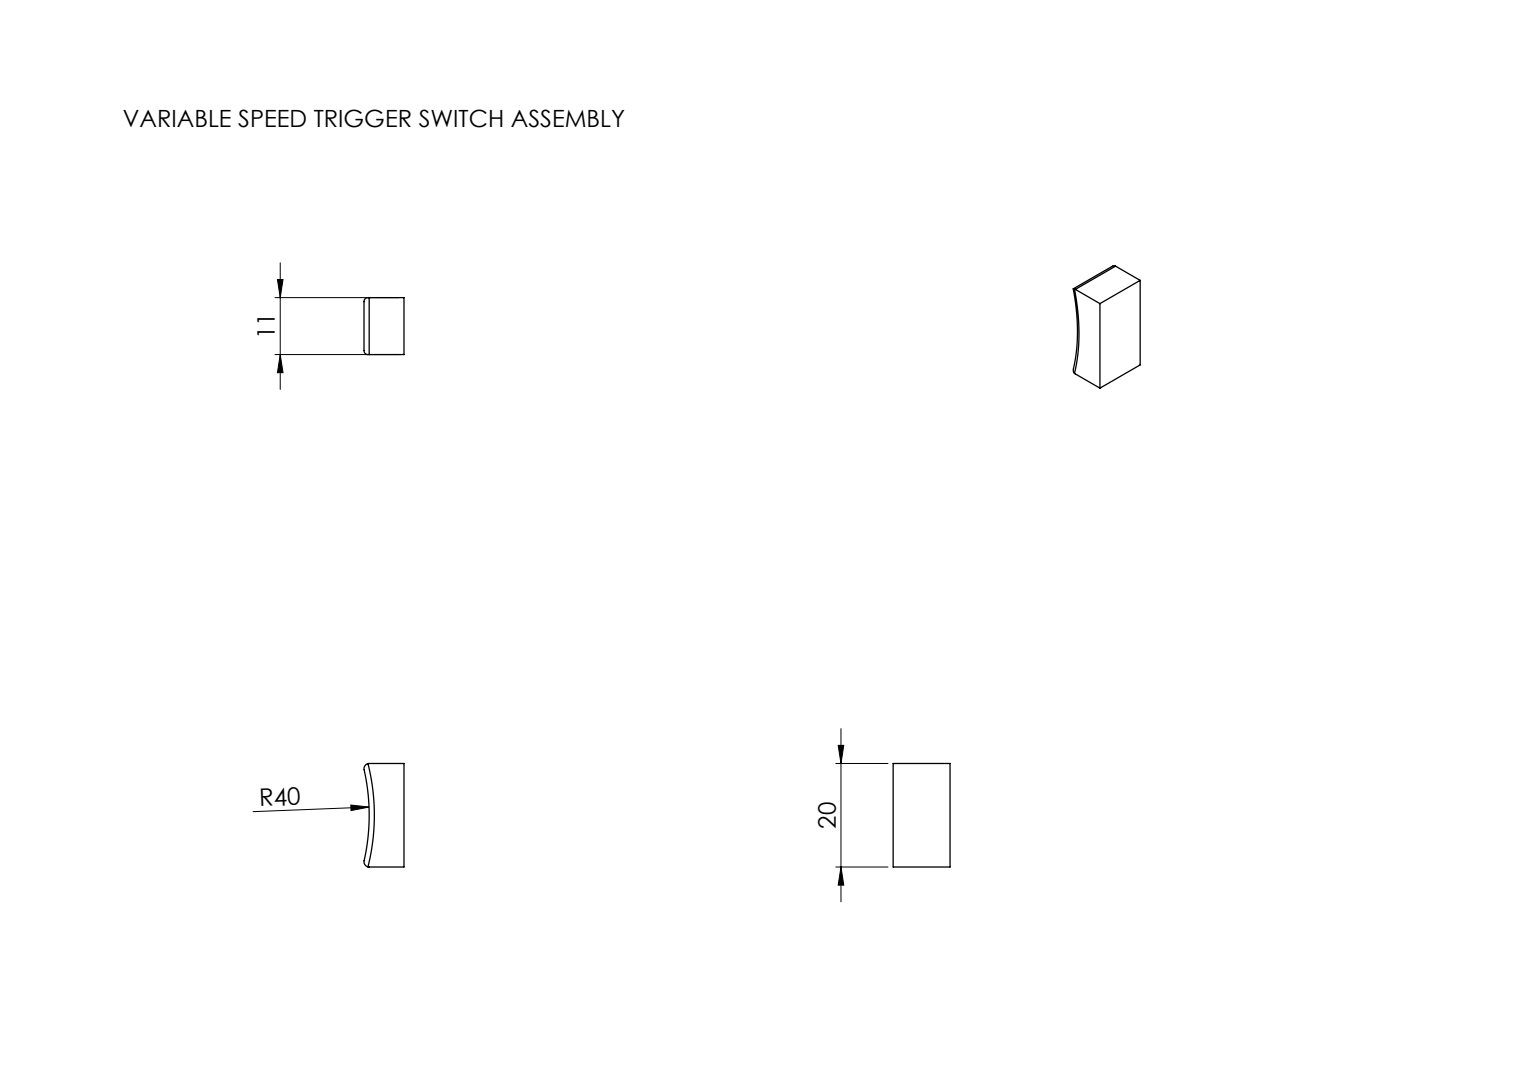
ISO-10303-21;
HEADER;
FILE_DESCRIPTION (('STEP AP214'),
    '1' );
FILE_NAME ('Variable Speed Trigger Switch assembly.step',
    '2026-10-05T20:22:16',
    ( '' ),
    ( '' ),
    'SwSTEP 2.0',
    'SolidWorks 2026',
    '' );
FILE_SCHEMA (( 'AUTOMOTIVE_DESIGN' ));
ENDSEC;

DATA;
#2=EDGE_CURVE ( 'NONE', #9188, #6176, #1844, .T. ) ;
#111=LINE ( 'NONE', #8166, #1932 ) ;
#145=DIRECTION ( 'NONE',  ( 0.000000000000000000, -0.000000000000000000, -1.000000000000000000 ) ) ;
#155=EDGE_CURVE ( 'NONE', #4227, #5635, #15763, .T. ) ;
#178=ORIENTED_EDGE ( 'NONE', *, *, #2632, .F. ) ;
#200=AXIS2_PLACEMENT_3D ( 'NONE', #10939, #4055, #145 ) ;
#265=DIRECTION ( 'NONE',  ( -0.000000000000000000, -0.000000000000000000, -1.000000000000000000 ) ) ;
#273=VECTOR ( 'NONE', #8822, 1000.000000000000000 ) ;
#311=CARTESIAN_POINT ( 'NONE',  ( -32.66708739526796279, 119.0000000000141824, -4.722170599054655860 ) ) ;
#314=CARTESIAN_POINT ( 'NONE',  ( -31.89848094669885725, 100.0271397714182342, 5.500000000000000000 ) ) ;
#331=CARTESIAN_POINT ( 'NONE',  ( -31.66708739526795924, 120.0000000000000284, -5.500000000000000000 ) ) ;
#383=DIRECTION ( 'NONE',  ( 3.469446951953614189E-16, -1.000000000000000000, 0.000000000000000000 ) ) ;
#427=VECTOR ( 'NONE', #13768, 1000.000000000000000 ) ;
#450=CARTESIAN_POINT ( 'NONE',  ( -32.02886766642249228, 119.9418479153533781, 5.500000000000000888 ) ) ;
#462=ORIENTED_EDGE ( 'NONE', *, *, #5545, .F. ) ;
#521=FILL_AREA_STYLE_COLOUR ( '', #2206 ) ;
#528=ORIENTED_EDGE ( 'NONE', *, *, #5545, .T. ) ;
#601=B_SPLINE_CURVE_WITH_KNOTS ( 'NONE', 3,
 ( #15955, #13311, #9052, #1176 ),
 .UNSPECIFIED., .F., .F.,
 ( 4, 4 ),
 ( -6.324563032106999871E-06, 0.0003067249959486805411 ),
 .UNSPECIFIED. ) ;
#623=EDGE_CURVE ( 'NONE', #8295, #4586, #6392, .T. ) ;
#656=CYLINDRICAL_SURFACE ( 'NONE', #15299, 1.000000000000000888 ) ;
#696=( LENGTH_UNIT ( ) NAMED_UNIT ( * ) SI_UNIT ( .MILLI., .METRE. ) );
#733=CARTESIAN_POINT ( 'NONE',  ( -32.64269715136552463, 118.7804878048780779, 4.500000000000000000 ) ) ;
#764=ORIENTED_EDGE ( 'NONE', *, *, #8937, .T. ) ;
#782=ADVANCED_FACE ( 'NONE', ( #2094 ), #7493, .T. ) ;
#907=CARTESIAN_POINT ( 'NONE',  ( -32.66708739526796279, 119.0000000000000284, 4.722170599040653727 ) ) ;
#1034=( NAMED_UNIT ( * ) SI_UNIT ( $, .STERADIAN. ) SOLID_ANGLE_UNIT ( ) );
#1168=DIRECTION ( 'NONE',  ( -1.000000000000000000, 0.000000000000000000, 0.000000000000000000 ) ) ;
#1176=CARTESIAN_POINT ( 'NONE',  ( -32.66708739526796279, 101.0000000000000142, 4.722170599040663497 ) ) ;
#1214=ADVANCED_FACE ( 'NONE', ( #11195 ), #11869, .T. ) ;
#1336=CARTESIAN_POINT ( 'NONE',  ( -71.66708739526794147, 110.0000000000000142, -4.499999999999999112 ) ) ;
#1469=VECTOR ( 'NONE', #5604, 1000.000000000000000 ) ;
#1494=PRODUCT ( 'Variable Speed Trigger Switch assembly', 'Variable Speed Trigger Switch assembly', '', ( #6686 ) ) ;
#1500=CARTESIAN_POINT ( 'NONE',  ( -32.59761674097325823, 119.3792650757663978, -5.080178642870992967 ) ) ;
#1501=CARTESIAN_POINT ( 'NONE',  ( -71.66708739526794147, 110.0000000000000142, -5.500000000000000000 ) ) ;
#1570=DIRECTION ( 'NONE',  ( 0.000000000000000000, 0.000000000000000000, 1.000000000000000000 ) ) ;
#1620=STYLED_ITEM ( 'NONE', ( #7941 ), #16900 ) ;
#1644=CARTESIAN_POINT ( 'NONE',  ( -32.02886766642248517, 100.0581520846466930, 5.500000000000000000 ) ) ;
#1692=ORIENTED_EDGE ( 'NONE', *, *, #9652, .F. ) ;
#1792=EDGE_LOOP ( 'NONE', ( #8992, #15963, #14025, #11089 ) ) ;
#1840=ORIENTED_EDGE ( 'NONE', *, *, #2784, .F. ) ;
#1842=EDGE_LOOP ( 'NONE', ( #6707, #13226, #11700, #4645 ) ) ;
#1844=B_SPLINE_CURVE_WITH_KNOTS ( 'NONE', 3,
 ( #8174, #11087, #2865, #16587 ),
 .UNSPECIFIED., .F., .F.,
 ( 4, 4 ),
 ( 0.001580575003428885293, 0.001893147295999754844 ),
 .UNSPECIFIED. ) ;
#1849=CARTESIAN_POINT ( 'NONE',  ( -31.66708739526795924, 119.0000000000000284, 5.500000000000000000 ) ) ;
#1853=AXIS2_PLACEMENT_3D ( 'NONE', #13518, #6796, #12191 ) ;
#1932=VECTOR ( 'NONE', #6853, 1000.000000000000000 ) ;
#1941=DIRECTION ( 'NONE',  ( -0.000000000000000000, -0.000000000000000000, -1.000000000000000000 ) ) ;
#1964=CARTESIAN_POINT ( 'NONE',  ( -32.14917720409752633, 119.8847850876495471, 5.472305571546614900 ) ) ;
#1979=EDGE_CURVE ( 'NONE', #5635, #9188, #7587, .T. ) ;
#2047=CARTESIAN_POINT ( 'NONE',  ( -31.66708739526795924, 101.0000000000000142, 5.500000000000000000 ) ) ;
#2094=FACE_OUTER_BOUND ( 'NONE', #9674, .T. ) ;
#2099=( NAMED_UNIT ( * ) SI_UNIT ( $, .STERADIAN. ) SOLID_ANGLE_UNIT ( ) );
#2113=VECTOR ( 'NONE', #4048, 1000.000000000000000 ) ;
#2140=CIRCLE ( 'NONE', #1853, 39.99999999999997868 ) ;
#2144=VERTEX_POINT ( 'NONE', #4204 ) ;
#2186=DIRECTION ( 'NONE',  ( -0.000000000000000000, -0.000000000000000000, -1.000000000000000000 ) ) ;
#2206=COLOUR_RGB ( '', 0.40784314, 0.44705882, 0.49803922) ;
#2370=PLANE ( 'NONE',  #14682 ) ;
#2381=CARTESIAN_POINT ( 'NONE',  ( -31.89848094669885725, 100.0271397714182342, -5.500000000000000000 ) ) ;
#2404=ORIENTED_EDGE ( 'NONE', *, *, #2, .F. ) ;
#2580=APPLICATION_CONTEXT ( 'automotive_design' ) ;
#2629=ORIENTED_EDGE ( 'NONE', *, *, #12849, .F. ) ;
#2632=EDGE_CURVE ( 'NONE', #7206, #9188, #16191, .T. ) ;
#2668=CARTESIAN_POINT ( 'NONE',  ( -71.66708739526794147, 110.0000000000000142, 4.500000000000000000 ) ) ;
#2744=CARTESIAN_POINT ( 'NONE',  ( -32.34996859904739352, 119.7408970890944744, -5.378151393595213214 ) ) ;
#2759=DIRECTION ( 'NONE',  ( 0.000000000000000000, 0.000000000000000000, 1.000000000000000000 ) ) ;
#2784=EDGE_CURVE ( 'NONE', #15700, #10662, #3443, .T. ) ;
#2785=ORIENTED_EDGE ( 'NONE', *, *, #1979, .T. ) ;
#2828=CARTESIAN_POINT ( 'NONE',  ( -32.66708739526796279, 119.0000000000141824, -4.722170599054655860 ) ) ;
#2833=DIRECTION ( 'NONE',  ( -1.000000000000000000, 0.000000000000000000, 0.000000000000000000 ) ) ;
#2865=CARTESIAN_POINT ( 'NONE',  ( -32.65876937324898677, 118.8519199021378938, -4.574127464417287570 ) ) ;
#2958=DIRECTION ( 'NONE',  ( -0.000000000000000000, -0.000000000000000000, -1.000000000000000000 ) ) ;
#3083=DIRECTION ( 'NONE',  ( -1.000000000000000000, 0.000000000000000000, 0.000000000000000000 ) ) ;
#3159=ORIENTED_EDGE ( 'NONE', *, *, #12950, .T. ) ;
#3179=( NAMED_UNIT ( * ) SI_UNIT ( $, .STERADIAN. ) SOLID_ANGLE_UNIT ( ) );
#3275=VERTEX_POINT ( 'NONE', #3762 ) ;
#3285=EDGE_CURVE ( 'NONE', #4393, #17452, #16707, .T. ) ;
#3290=LINE ( 'NONE', #14101, #1469 ) ;
#3291=CARTESIAN_POINT ( 'NONE',  ( -32.34996859905196231, 119.7408970890905096, 5.378151393592371043 ) ) ;
#3303=ORIENTED_EDGE ( 'NONE', *, *, #6295, .T. ) ;
#3441=SURFACE_SIDE_STYLE ('',( #15381 ) ) ;
#3443=LINE ( 'NONE', #14238, #11031 ) ;
#3473=CARTESIAN_POINT ( 'NONE',  ( -32.66708739526796279, 118.9256726598784866, 4.648823768412006174 ) ) ;
#3475=VERTEX_POINT ( 'NONE', #11444 ) ;
#3476=ADVANCED_FACE ( 'NONE', ( #11180 ), #16854, .F. ) ;
#3480=ORIENTED_EDGE ( 'NONE', *, *, #10562, .F. ) ;
#3518=CARTESIAN_POINT ( 'NONE',  ( -32.66708739526796279, 119.0000000000000284, 5.500000000000000000 ) ) ;
#3583=AXIS2_PLACEMENT_3D ( 'NONE', #5482, #6893, #8222 ) ;
#3762=CARTESIAN_POINT ( 'NONE',  ( -24.93725393319378725, 100.0000000000000142, 5.500000000000000000 ) ) ;
#3768=CARTESIAN_POINT ( 'NONE',  ( -32.66708739526796279, 101.0000000000000142, -4.722170599040662609 ) ) ;
#3776=FILL_AREA_STYLE_COLOUR ( '', #15186 ) ;
#3789=UNCERTAINTY_MEASURE_WITH_UNIT (LENGTH_MEASURE( 1.000000000000000082E-05 ), #696, 'distance_accuracy_value', 'NONE');
#3800=EDGE_CURVE ( 'NONE', #17452, #7206, #7303, .T. ) ;
#3887=( GEOMETRIC_REPRESENTATION_CONTEXT ( 3 ) GLOBAL_UNCERTAINTY_ASSIGNED_CONTEXT ( ( #17305 ) ) GLOBAL_UNIT_ASSIGNED_CONTEXT ( ( #11826, #10317, #1034 ) ) REPRESENTATION_CONTEXT ( 'NONE', 'WORKASPACE' ) );
#3915=ORIENTED_EDGE ( 'NONE', *, *, #623, .T. ) ;
#3973=CARTESIAN_POINT ( 'NONE',  ( -32.43085388486576193, 100.3453498474263910, -5.312352690998809912 ) ) ;
#4048=DIRECTION ( 'NONE',  ( -1.000000000000000000, -0.000000000000000000, -0.000000000000000000 ) ) ;
#4055=DIRECTION ( 'NONE',  ( 0.000000000000000000, -1.000000000000000000, 0.000000000000000000 ) ) ;
#4103=CARTESIAN_POINT ( 'NONE',  ( -31.89848094669886436, 119.9728602285818084, -5.500000000000000000 ) ) ;
#4117=CARTESIAN_POINT ( 'NONE',  ( -32.66708739526796279, 119.0000000000000284, 4.722170599040653727 ) ) ;
#4204=CARTESIAN_POINT ( 'NONE',  ( -24.93725393319379435, 120.0000000000000284, -5.500000000000000000 ) ) ;
#4227=VERTEX_POINT ( 'NONE', #7143 ) ;
#4249=CARTESIAN_POINT ( 'NONE',  ( -32.55406425504222057, 119.4745293701363664, -5.163900856529947347 ) ) ;
#4276=CARTESIAN_POINT ( 'NONE',  ( -32.64269715136552463, 118.7804878048780779, -4.499999999999999112 ) ) ;
#4297=CARTESIAN_POINT ( 'NONE',  ( -71.66708739526794147, 110.0000000000000142, 5.500000000000000000 ) ) ;
#4322=LINE ( 'NONE', #13700, #7340 ) ;
#4324=CARTESIAN_POINT ( 'NONE',  ( -32.64269715136552463, 101.2195121951219647, -4.499999999999999112 ) ) ;
#4332=DIRECTION ( 'NONE',  ( 0.000000000000000000, 0.000000000000000000, 1.000000000000000000 ) ) ;
#4379=DIRECTION ( 'NONE',  ( -0.000000000000000000, -0.000000000000000000, -1.000000000000000000 ) ) ;
#4393=VERTEX_POINT ( 'NONE', #11387 ) ;
#4452=CARTESIAN_POINT ( 'NONE',  ( -32.66708739526796279, 119.0000000000000284, 4.722170599040653727 ) ) ;
#4475=CARTESIAN_POINT ( 'NONE',  ( -31.66708739526795924, 101.0000000000000142, 5.500000000000000000 ) ) ;
#4477=PRODUCT_DEFINITION_SHAPE ( 'NONE', 'NONE',  #5120 ) ;
#4508=CARTESIAN_POINT ( 'NONE',  ( -71.66708739526794147, 110.0000000000000142, -5.500000000000000000 ) ) ;
#4586=VERTEX_POINT ( 'NONE', #9419 ) ;
#4627=CARTESIAN_POINT ( 'NONE',  ( -32.43085388486576193, 119.6546501525736375, 5.312352690998810800 ) ) ;
#4645=ORIENTED_EDGE ( 'NONE', *, *, #8937, .F. ) ;
#4727=VECTOR ( 'NONE', #265, 1000.000000000000000 ) ;
#4734=ORIENTED_EDGE ( 'NONE', *, *, #12950, .F. ) ;
#4735=CARTESIAN_POINT ( 'NONE',  ( -32.43085388486576903, 100.3453498474263768, 5.312352690998809024 ) ) ;
#4772=SHAPE_REPRESENTATION_RELATIONSHIP ( 'NONE' , 'NONE' ,  #13460, #10572 ) ;
#4829=AXIS2_PLACEMENT_3D ( 'NONE', #11999, #14921, #8191 ) ;
#4833=AXIS2_PLACEMENT_3D ( 'NONE', #14393, #17123, #5002 ) ;
#4933=DIRECTION ( 'NONE',  ( -0.000000000000000000, -0.000000000000000000, -1.000000000000000000 ) ) ;
#4972=CARTESIAN_POINT ( 'NONE',  ( -71.66708739526794147, 110.0000000000000142, 4.500000000000000000 ) ) ;
#5002=DIRECTION ( 'NONE',  ( -1.000000000000000000, 0.000000000000000000, 0.000000000000000000 ) ) ;
#5009=LINE ( 'NONE', #17132, #2113 ) ;
#5018=CARTESIAN_POINT ( 'NONE',  ( -31.89848094669885725, 100.0271397714182342, -5.500000000000000000 ) ) ;
#5120=PRODUCT_DEFINITION ( 'UNKNOWN', '', #12096, #9369 ) ;
#5288=SURFACE_STYLE_FILL_AREA ( #6263 ) ;
#5482=CARTESIAN_POINT ( 'NONE',  ( 0.000000000000000000, 0.000000000000000000, 0.000000000000000000 ) ) ;
#5515=EDGE_LOOP ( 'NONE', ( #5570, #16193, #16050, #7766, #14975, #16631 ) ) ;
#5545=EDGE_CURVE ( 'NONE', #17341, #4393, #12084, .T. ) ;
#5570=ORIENTED_EDGE ( 'NONE', *, *, #6017, .T. ) ;
#5604=DIRECTION ( 'NONE',  ( 1.000000000000000000, -0.000000000000000000, -0.000000000000000000 ) ) ;
#5635=VERTEX_POINT ( 'NONE', #4117 ) ;
#5638=ADVANCED_FACE ( 'NONE', ( #6784 ), #8350, .F. ) ;
#5713=DIRECTION ( 'NONE',  ( -1.000000000000000000, 0.000000000000000000, 0.000000000000000000 ) ) ;
#5725=ORIENTED_EDGE ( 'NONE', *, *, #8449, .T. ) ;
#5741=ORIENTED_EDGE ( 'NONE', *, *, #3800, .F. ) ;
#5780=VECTOR ( 'NONE', #8506, 1000.000000000000000 ) ;
#5782=CARTESIAN_POINT ( 'NONE',  ( -31.66708739526795924, 100.0000000000000142, 5.500000000000000000 ) ) ;
#5836=DIRECTION ( 'NONE',  ( -1.000000000000000000, 0.000000000000000000, 0.000000000000000000 ) ) ;
#5845=DIRECTION ( 'NONE',  ( -0.000000000000000000, -0.000000000000000000, -1.000000000000000000 ) ) ;
#5855=CARTESIAN_POINT ( 'NONE',  ( -32.66708739526796279, 101.0000000000000142, -4.722170599040662609 ) ) ;
#5859=TOROIDAL_SURFACE ( 'NONE', #8394, 40.99999999999998579, 1.000000000000000000 ) ;
#5902=ORIENTED_EDGE ( 'NONE', *, *, #3800, .T. ) ;
#5952=CARTESIAN_POINT ( 'NONE',  ( -32.64269715136552463, 101.2195121951219647, -4.499999999999999112 ) ) ;
#5980=CARTESIAN_POINT ( 'NONE',  ( -32.59761674097720174, 100.6207349242430809, 5.080178642862614780 ) ) ;
#6009=( LENGTH_UNIT ( ) NAMED_UNIT ( * ) SI_UNIT ( .MILLI., .METRE. ) );
#6017=EDGE_CURVE ( 'NONE', #11430, #3475, #601, .T. ) ;
#6111=ORIENTED_EDGE ( 'NONE', *, *, #8449, .F. ) ;
#6176=VERTEX_POINT ( 'NONE', #4276 ) ;
#6263=FILL_AREA_STYLE ('',( #3776 ) ) ;
#6265=EDGE_LOOP ( 'NONE', ( #8080, #14588, #3915, #3303, #5725, #8757 ) ) ;
#6295=EDGE_CURVE ( 'NONE', #4586, #17341, #14879, .T. ) ;
#6315=EDGE_LOOP ( 'NONE', ( #5902, #3159, #9035, #3480, #1692, #16838 ) ) ;
#6392=CIRCLE ( 'NONE', #7530, 40.99999999999997868 ) ;
#6499=ORIENTED_EDGE ( 'NONE', *, *, #6295, .F. ) ;
#6531=CARTESIAN_POINT ( 'NONE',  ( -32.14917720409751922, 100.1152149123505239, -5.472305571546616676 ) ) ;
#6638=VERTEX_POINT ( 'NONE', #8574 ) ;
#6640=CARTESIAN_POINT ( 'NONE',  ( -32.14917720409452073, 119.8847850876509966, -5.472305571547330771 ) ) ;
#6686=PRODUCT_CONTEXT ( 'NONE', #7328, 'mechanical' ) ;
#6707=ORIENTED_EDGE ( 'NONE', *, *, #14410, .F. ) ;
#6752=EDGE_CURVE ( 'NONE', #10662, #8295, #8594, .T. ) ;
#6784=FACE_OUTER_BOUND ( 'NONE', #14962, .T. ) ;
#6791=ORIENTED_EDGE ( 'NONE', *, *, #2, .T. ) ;
#6796=DIRECTION ( 'NONE',  ( -0.000000000000000000, -0.000000000000000000, -1.000000000000000000 ) ) ;
#6827=DIRECTION ( 'NONE',  ( -0.000000000000000000, -0.000000000000000000, -1.000000000000000000 ) ) ;
#6853=DIRECTION ( 'NONE',  ( -1.000000000000000000, -0.000000000000000000, -0.000000000000000000 ) ) ;
#6893=DIRECTION ( 'NONE',  ( 0.000000000000000000, 0.000000000000000000, 1.000000000000000000 ) ) ;
#6990=FACE_OUTER_BOUND ( 'NONE', #17295, .T. ) ;
#7054=CIRCLE ( 'NONE', #16949, 39.99999999999997868 ) ;
#7143=CARTESIAN_POINT ( 'NONE',  ( -32.64269715136552463, 118.7804878048780779, 4.500000000000000000 ) ) ;
#7169=ORIENTED_EDGE ( 'NONE', *, *, #11708, .F. ) ;
#7206=VERTEX_POINT ( 'NONE', #4103 ) ;
#7245=AXIS2_PLACEMENT_3D ( 'NONE', #2047, #7440, #12841 ) ;
#7250=DIRECTION ( 'NONE',  ( -1.000000000000000000, 0.000000000000000000, 0.000000000000000000 ) ) ;
#7298=CARTESIAN_POINT ( 'NONE',  ( -32.66708739526796279, 101.0000000000000142, 4.722170599040663497 ) ) ;
#7303=CIRCLE ( 'NONE', #14648, 40.99999999999997868 ) ;
#7328=APPLICATION_CONTEXT ( 'automotive_design' ) ;
#7340=VECTOR ( 'NONE', #1570, 1000.000000000000000 ) ;
#7402=ORIENTED_EDGE ( 'NONE', *, *, #16890, .T. ) ;
#7405=EDGE_CURVE ( 'NONE', #5635, #8295, #9583, .T. ) ;
#7440=DIRECTION ( 'NONE',  ( 0.000000000000000000, 0.000000000000000000, 1.000000000000000000 ) ) ;
#7493=CYLINDRICAL_SURFACE ( 'NONE', #13015, 1.000000000000000888 ) ;
#7530=AXIS2_PLACEMENT_3D ( 'NONE', #8767, #5845, #12925 ) ;
#7540=CARTESIAN_POINT ( 'NONE',  ( -32.65879391391307252, 118.8520289717560843, 4.574240649589675911 ) ) ;
#7587=LINE ( 'NONE', #3518, #16113 ) ;
#7671=CARTESIAN_POINT ( 'NONE',  ( -32.02886766642249228, 100.0581520846466645, -5.500000000000001776 ) ) ;
#7766=ORIENTED_EDGE ( 'NONE', *, *, #7405, .F. ) ;
#7930=VECTOR ( 'NONE', #15717, 1000.000000000000000 ) ;
#7941=PRESENTATION_STYLE_ASSIGNMENT (( #11654 ) ) ;
#7977=DIRECTION ( 'NONE',  ( -0.000000000000000000, -0.000000000000000000, -1.000000000000000000 ) ) ;
#8080=ORIENTED_EDGE ( 'NONE', *, *, #14108, .T. ) ;
#8120=CARTESIAN_POINT ( 'NONE',  ( -24.93725393319378725, 100.0000000000000142, 5.500000000000000000 ) ) ;
#8149=CARTESIAN_POINT ( 'NONE',  ( -32.66708739526796279, 101.0000000000000142, 5.500000000000000000 ) ) ;
#8166=CARTESIAN_POINT ( 'NONE',  ( -32.93725393319379435, 120.0000000000000284, 5.500000000000000000 ) ) ;
#8174=CARTESIAN_POINT ( 'NONE',  ( -32.66708739526796279, 119.0000000000141824, -4.722170599054655860 ) ) ;
#8191=DIRECTION ( 'NONE',  ( -1.000000000000000000, 0.000000000000000000, 0.000000000000000000 ) ) ;
#8222=DIRECTION ( 'NONE',  ( 1.000000000000000000, 0.000000000000000000, 0.000000000000000000 ) ) ;
#8223=CARTESIAN_POINT ( 'NONE',  ( -32.66708739526662697, 119.0939651702628623, -4.814896201988002389 ) ) ;
#8295=VERTEX_POINT ( 'NONE', #9709 ) ;
#8350=CYLINDRICAL_SURFACE ( 'NONE', #13454, 39.99999999999997868 ) ;
#8358=CARTESIAN_POINT ( 'NONE',  ( -32.34996859905195521, 100.2591029109095189, 5.378151393592374596 ) ) ;
#8365=EDGE_LOOP ( 'NONE', ( #11702, #13362, #11371, #15316, #462, #6499 ) ) ;
#8394=AXIS2_PLACEMENT_3D ( 'NONE', #1336, #1941, #5836 ) ;
#8419=FACE_OUTER_BOUND ( 'NONE', #14217, .T. ) ;
#8449=EDGE_CURVE ( 'NONE', #17341, #3275, #11565, .T. ) ;
#8450=FACE_OUTER_BOUND ( 'NONE', #1842, .T. ) ;
#8500=AXIS2_PLACEMENT_3D ( 'NONE', #16574, #4933, #12671 ) ;
#8506=DIRECTION ( 'NONE',  ( -3.469446951953613696E-16, 1.000000000000000000, -0.000000000000000000 ) ) ;
#8574=CARTESIAN_POINT ( 'NONE',  ( -24.93725393319378725, 100.0000000000000142, -5.500000000000000000 ) ) ;
#8594=CIRCLE ( 'NONE', #8865, 1.000000000000000888 ) ;
#8604=ADVANCED_FACE ( 'NONE', ( #9254 ), #13338, .F. ) ;
#8757=ORIENTED_EDGE ( 'NONE', *, *, #16378, .T. ) ;
#8767=CARTESIAN_POINT ( 'NONE',  ( -71.66708739526794147, 110.0000000000000142, 5.500000000000000000 ) ) ;
#8822=DIRECTION ( 'NONE',  ( -3.469446951953613696E-16, 1.000000000000000000, -0.000000000000000000 ) ) ;
#8865=AXIS2_PLACEMENT_3D ( 'NONE', #1849, #12481, #7250 ) ;
#8885=ADVANCED_FACE ( 'NONE', ( #8419 ), #15324, .T. ) ;
#8910=DIRECTION ( 'NONE',  ( -0.000000000000000000, -0.000000000000000000, 1.000000000000000000 ) ) ;
#8937=EDGE_CURVE ( 'NONE', #10732, #11377, #13716, .T. ) ;
#8992=ORIENTED_EDGE ( 'NONE', *, *, #10734, .T. ) ;
#9035=ORIENTED_EDGE ( 'NONE', *, *, #10734, .F. ) ;
#9052=CARTESIAN_POINT ( 'NONE',  ( -32.66708739526796279, 101.0743273401215419, 4.648823768412004398 ) ) ;
#9085=CARTESIAN_POINT ( 'NONE',  ( -32.55406425504676093, 100.5254706298718901, -5.163900856522908533 ) ) ;
#9112=EDGE_CURVE ( 'NONE', #15090, #2144, #12086, .T. ) ;
#9171=SURFACE_SIDE_STYLE ('',( #5288 ) ) ;
#9188=VERTEX_POINT ( 'NONE', #311 ) ;
#9235=ADVANCED_FACE ( 'NONE', ( #9947 ), #656, .T. ) ;
#9252=CARTESIAN_POINT ( 'NONE',  ( -31.66708739526795924, 120.0000000000000284, 5.500000000000000000 ) ) ;
#9254=FACE_OUTER_BOUND ( 'NONE', #6265, .T. ) ;
#9343=ORIENTED_EDGE ( 'NONE', *, *, #15326, .T. ) ;
#9369=PRODUCT_DEFINITION_CONTEXT ( 'detailed design', #2580, 'design' ) ;
#9419=CARTESIAN_POINT ( 'NONE',  ( -31.89848094669885725, 100.0271397714182342, 5.500000000000000000 ) ) ;
#9448=ORIENTED_EDGE ( 'NONE', *, *, #10562, .T. ) ;
#9551=CARTESIAN_POINT ( 'NONE',  ( -31.66708739526795924, 119.0000000000000284, -5.500000000000000000 ) ) ;
#9583=B_SPLINE_CURVE_WITH_KNOTS ( 'NONE', 3,
 ( #4452, #14102, #10191, #15244, #15331, #4627, #3291, #1964, #450, #14189 ),
 .UNSPECIFIED., .F., .F.,
 ( 4, 2, 2, 2, 4 ),
 ( 0.0003067249959486639528, 0.0007024845516937828528, 0.001098244107438901915, 0.001494003663184020761, 0.001889763218929139824 ),
 .UNSPECIFIED. ) ;
#9645=ORIENTED_EDGE ( 'NONE', *, *, #15326, .F. ) ;
#9652=EDGE_CURVE ( 'NONE', #4393, #6638, #3290, .T. ) ;
#9674=EDGE_LOOP ( 'NONE', ( #17183, #11314, #16308, #1840, #4734, #10382 ) ) ;
#9709=CARTESIAN_POINT ( 'NONE',  ( -31.89848094669886436, 119.9728602285818084, 5.500000000000000000 ) ) ;
#9710=B_SPLINE_CURVE_WITH_KNOTS ( 'NONE', 3,
 ( #7298, #16864, #13774, #5980, #11372, #4735, #8358, #13871, #1644, #314 ),
 .UNSPECIFIED., .F., .F.,
 ( 4, 2, 2, 2, 4 ),
 ( 0.0003067249959486805411, 0.0007024845516937958632, 0.001098244107438911240, 0.001494003663184026399, 0.001889763218929141775 ),
 .UNSPECIFIED. ) ;
#9783=CLOSED_SHELL ( 'NONE', ( #8885, #9235, #5638, #10274, #3476, #17019, #8604, #16849, #12631, #1214, #13022, #782 ) ) ;
#9837=( GEOMETRIC_REPRESENTATION_CONTEXT ( 3 ) GLOBAL_UNCERTAINTY_ASSIGNED_CONTEXT ( ( #16009 ) ) GLOBAL_UNIT_ASSIGNED_CONTEXT ( ( #6009, #12998, #3179 ) ) REPRESENTATION_CONTEXT ( 'NONE', 'WORKASPACE' ) );
#9947=FACE_OUTER_BOUND ( 'NONE', #8365, .T. ) ;
#10020=CARTESIAN_POINT ( 'NONE',  ( -24.93725393319379435, 120.0000000000000284, 5.500000000000000000 ) ) ;
#10088=MECHANICAL_DESIGN_GEOMETRIC_PRESENTATION_REPRESENTATION('',(#1620),#3887);
#10191=CARTESIAN_POINT ( 'NONE',  ( -32.65377812985507688, 119.1901795341116923, 4.906772862994290385 ) ) ;
#10274=ADVANCED_FACE ( 'NONE', ( #17423 ), #2370, .F. ) ;
#10313=EDGE_CURVE ( 'NONE', #11377, #11430, #4322, .T. ) ;
#10317=( NAMED_UNIT ( * ) PLANE_ANGLE_UNIT ( ) SI_UNIT ( $, .RADIAN. ) );
#10382=ORIENTED_EDGE ( 'NONE', *, *, #2632, .T. ) ;
#10410=CARTESIAN_POINT ( 'NONE',  ( -32.66708739526796279, 101.0000000000000142, -4.722170599040662609 ) ) ;
#10562=EDGE_CURVE ( 'NONE', #6638, #2144, #11473, .T. ) ;
#10572=ADVANCED_BREP_SHAPE_REPRESENTATION ( '', ( #16900, #3583 ), #9837 ) ;
#10660=CIRCLE ( 'NONE', #14072, 1.000000000000000888 ) ;
#10662=VERTEX_POINT ( 'NONE', #9252 ) ;
#10732=VERTEX_POINT ( 'NONE', #3768 ) ;
#10734=EDGE_CURVE ( 'NONE', #2144, #15700, #5009, .T. ) ;
#10759=DIRECTION ( 'NONE',  ( -1.000000000000000000, 0.000000000000000000, 0.000000000000000000 ) ) ;
#10836=SHAPE_DEFINITION_REPRESENTATION ( #4477, #13460 ) ;
#10939=CARTESIAN_POINT ( 'NONE',  ( -32.93725393319379435, 120.0000000000000284, 5.500000000000000000 ) ) ;
#10940=ORIENTED_EDGE ( 'NONE', *, *, #11708, .T. ) ;
#10964=CARTESIAN_POINT ( 'NONE',  ( -32.65377812985267525, 119.1901795341236578, -4.906772863005508079 ) ) ;
#11031=VECTOR ( 'NONE', #8910, 1000.000000000000000 ) ;
#11087=CARTESIAN_POINT ( 'NONE',  ( -32.66708739526901439, 118.9256703196821263, -4.648821459087186803 ) ) ;
#11089=ORIENTED_EDGE ( 'NONE', *, *, #9112, .T. ) ;
#11115=PLANE ( 'NONE',  #200 ) ;
#11136=LINE ( 'NONE', #15121, #4727 ) ;
#11147=LINE ( 'NONE', #16566, #5780 ) ;
#11180=FACE_OUTER_BOUND ( 'NONE', #17058, .T. ) ;
#11195=FACE_OUTER_BOUND ( 'NONE', #5515, .T. ) ;
#11221=FACE_OUTER_BOUND ( 'NONE', #6315, .T. ) ;
#11314=ORIENTED_EDGE ( 'NONE', *, *, #7405, .T. ) ;
#11368=CARTESIAN_POINT ( 'NONE',  ( -31.66708739526795924, 101.0000000000000142, 5.500000000000000000 ) ) ;
#11371=ORIENTED_EDGE ( 'NONE', *, *, #16890, .F. ) ;
#11372=CARTESIAN_POINT ( 'NONE',  ( -32.55406425504675383, 100.5254706298719185, 5.163900856522908533 ) ) ;
#11377=VERTEX_POINT ( 'NONE', #4324 ) ;
#11387=CARTESIAN_POINT ( 'NONE',  ( -31.66708739526795924, 100.0000000000000142, -5.500000000000000000 ) ) ;
#11430=VERTEX_POINT ( 'NONE', #13628 ) ;
#11444=CARTESIAN_POINT ( 'NONE',  ( -32.66708739526796279, 101.0000000000000142, 4.722170599040663497 ) ) ;
#11473=LINE ( 'NONE', #17050, #273 ) ;
#11486=PRESENTATION_STYLE_ASSIGNMENT (( #15644 ) ) ;
#11508=AXIS2_PLACEMENT_3D ( 'NONE', #4508, #15302, #15564 ) ;
#11565=LINE ( 'NONE', #12813, #7930 ) ;
#11575=FILL_AREA_STYLE ('',( #521 ) ) ;
#11627=VECTOR ( 'NONE', #13600, 1000.000000000000000 ) ;
#11654=SURFACE_STYLE_USAGE ( .BOTH. , #9171 ) ;
#11700=ORIENTED_EDGE ( 'NONE', *, *, #10313, .F. ) ;
#11702=ORIENTED_EDGE ( 'NONE', *, *, #13896, .F. ) ;
#11708=EDGE_CURVE ( 'NONE', #6176, #11377, #2140, .T. ) ;
#11733=CARTESIAN_POINT ( 'NONE',  ( -32.66708739526796990, 100.9060348297503964, -4.814896201975306766 ) ) ;
#11826=( LENGTH_UNIT ( ) NAMED_UNIT ( * ) SI_UNIT ( .MILLI., .METRE. ) );
#11869=TOROIDAL_SURFACE ( 'NONE', #14149, 40.99999999999998579, 1.000000000000000000 ) ;
#11872=DIRECTION ( 'NONE',  ( -0.000000000000000000, -0.000000000000000000, -1.000000000000000000 ) ) ;
#11918=CARTESIAN_POINT ( 'NONE',  ( -32.59761674097722306, 100.6207349242431093, -5.080178642862613003 ) ) ;
#11999=CARTESIAN_POINT ( 'NONE',  ( -71.66708739526794147, 110.0000000000000142, 5.500000000000000000 ) ) ;
#12033=CARTESIAN_POINT ( 'NONE',  ( -31.89848094669886436, 119.9728602285818084, -5.500000000000000000 ) ) ;
#12084=LINE ( 'NONE', #15170, #427 ) ;
#12086=LINE ( 'NONE', #13509, #11627 ) ;
#12096=PRODUCT_DEFINITION_FORMATION_WITH_SPECIFIED_SOURCE ( 'ANY', '', #1494, .NOT_KNOWN. ) ;
#12110=STYLED_ITEM ( 'NONE', ( #11486 ), #10572 ) ;
#12191=DIRECTION ( 'NONE',  ( -1.000000000000000000, 0.000000000000000000, 0.000000000000000000 ) ) ;
#12386=CARTESIAN_POINT ( 'NONE',  ( -32.43085388486101550, 119.6546501525790234, -5.312352691002971028 ) ) ;
#12441=CYLINDRICAL_SURFACE ( 'NONE', #15168, 1.000000000000000888 ) ;
#12481=DIRECTION ( 'NONE',  ( 0.000000000000000000, 0.000000000000000000, 1.000000000000000000 ) ) ;
#12631=ADVANCED_FACE ( 'NONE', ( #8450 ), #12441, .T. ) ;
#12671=DIRECTION ( 'NONE',  ( -1.000000000000000000, 0.000000000000000000, 0.000000000000000000 ) ) ;
#12775=CARTESIAN_POINT ( 'NONE',  ( -24.93725393319379435, 120.0000000000000284, 5.500000000000000000 ) ) ;
#12813=CARTESIAN_POINT ( 'NONE',  ( -24.93725393319378725, 100.0000000000000142, 5.500000000000000000 ) ) ;
#12841=DIRECTION ( 'NONE',  ( -1.000000000000000000, 0.000000000000000000, 0.000000000000000000 ) ) ;
#12849=EDGE_CURVE ( 'NONE', #4227, #6176, #11136, .T. ) ;
#12925=DIRECTION ( 'NONE',  ( -1.000000000000000000, 0.000000000000000000, 0.000000000000000000 ) ) ;
#12950=EDGE_CURVE ( 'NONE', #7206, #15700, #10660, .T. ) ;
#12998=( NAMED_UNIT ( * ) PLANE_ANGLE_UNIT ( ) SI_UNIT ( $, .RADIAN. ) );
#13015=AXIS2_PLACEMENT_3D ( 'NONE', #15206, #14068, #3083 ) ;
#13022=ADVANCED_FACE ( 'NONE', ( #6990 ), #5859, .T. ) ;
#13031=AXIS2_PLACEMENT_3D ( 'NONE', #10020, #16773, #383 ) ;
#13037=CARTESIAN_POINT ( 'NONE',  ( -24.93725393319378725, 100.0000000000000142, 5.500000000000000000 ) ) ;
#13041=DIRECTION ( 'NONE',  ( -1.000000000000000000, 0.000000000000000000, 0.000000000000000000 ) ) ;
#13088=ORIENTED_EDGE ( 'NONE', *, *, #9652, .T. ) ;
#13203=LINE ( 'NONE', #13037, #14684 ) ;
#13213=ORIENTED_EDGE ( 'NONE', *, *, #10313, .T. ) ;
#13226=ORIENTED_EDGE ( 'NONE', *, *, #6017, .F. ) ;
#13311=CARTESIAN_POINT ( 'NONE',  ( -32.65879391391417386, 101.1479710282390840, 4.574240649584753626 ) ) ;
#13318=ORIENTED_EDGE ( 'NONE', *, *, #16378, .F. ) ;
#13338=PLANE ( 'NONE',  #4829 ) ;
#13362=ORIENTED_EDGE ( 'NONE', *, *, #14410, .T. ) ;
#13367=CARTESIAN_POINT ( 'NONE',  ( -32.02886766642084382, 119.9418479153537334, -5.500000000000000000 ) ) ;
#13454=AXIS2_PLACEMENT_3D ( 'NONE', #4297, #4379, #10759 ) ;
#13460=SHAPE_REPRESENTATION ( 'Variable Speed Trigger Switch assembly', ( #3583 ), #9837 ) ;
#13487=MECHANICAL_DESIGN_GEOMETRIC_PRESENTATION_REPRESENTATION('',(#12110),#14367);
#13509=CARTESIAN_POINT ( 'NONE',  ( -24.93725393319379435, 120.0000000000000284, 5.500000000000000000 ) ) ;
#13518=CARTESIAN_POINT ( 'NONE',  ( -71.66708739526794147, 110.0000000000000142, -4.499999999999999112 ) ) ;
#13532=DIRECTION ( 'NONE',  ( 0.000000000000000000, 1.000000000000000000, -0.000000000000000000 ) ) ;
#13600=DIRECTION ( 'NONE',  ( -0.000000000000000000, -0.000000000000000000, -1.000000000000000000 ) ) ;
#13628=CARTESIAN_POINT ( 'NONE',  ( -32.64269715136552463, 101.2195121951219647, 4.500000000000000000 ) ) ;
#13700=CARTESIAN_POINT ( 'NONE',  ( -32.64269715136551753, 101.2195121951219647, 5.500000000000000000 ) ) ;
#13716=B_SPLINE_CURVE_WITH_KNOTS ( 'NONE', 3,
 ( #5855, #13738, #13922, #5952 ),
 .UNSPECIFIED., .F., .F.,
 ( 4, 4 ),
 ( 0.001580575003448743973, 0.001893147295999755278 ),
 .UNSPECIFIED. ) ;
#13738=CARTESIAN_POINT ( 'NONE',  ( -32.66708739526796279, 101.0743296803272386, -4.648821459077780993 ) ) ;
#13768=DIRECTION ( 'NONE',  ( 0.000000000000000000, 0.000000000000000000, -1.000000000000000000 ) ) ;
#13774=CARTESIAN_POINT ( 'NONE',  ( -32.65377812985507688, 100.8098204658883645, 4.906772862994293050 ) ) ;
#13871=CARTESIAN_POINT ( 'NONE',  ( -32.14917720409751922, 100.1152149123505382, 5.472305571546616676 ) ) ;
#13896=EDGE_CURVE ( 'NONE', #3475, #4586, #9710, .T. ) ;
#13922=CARTESIAN_POINT ( 'NONE',  ( -32.65876937324905072, 101.1480800978618362, -4.574127464407660604 ) ) ;
#13980=( NAMED_UNIT ( * ) PLANE_ANGLE_UNIT ( ) SI_UNIT ( $, .RADIAN. ) );
#14025=ORIENTED_EDGE ( 'NONE', *, *, #14108, .F. ) ;
#14033=DIRECTION ( 'NONE',  ( -1.000000000000000000, 0.000000000000000000, 0.000000000000000000 ) ) ;
#14068=DIRECTION ( 'NONE',  ( -0.000000000000000000, -0.000000000000000000, -1.000000000000000000 ) ) ;
#14072=AXIS2_PLACEMENT_3D ( 'NONE', #9551, #6827, #2833 ) ;
#14101=CARTESIAN_POINT ( 'NONE',  ( -24.93725393319378725, 100.0000000000000142, -5.500000000000000000 ) ) ;
#14102=CARTESIAN_POINT ( 'NONE',  ( -32.66708739526796990, 119.0939651702496178, 4.814896201975304102 ) ) ;
#14108=EDGE_CURVE ( 'NONE', #15090, #10662, #111, .T. ) ;
#14149=AXIS2_PLACEMENT_3D ( 'NONE', #4972, #15187, #13041 ) ;
#14179=ORIENTED_EDGE ( 'NONE', *, *, #155, .T. ) ;
#14189=CARTESIAN_POINT ( 'NONE',  ( -31.89848094669886436, 119.9728602285818084, 5.500000000000000000 ) ) ;
#14217=EDGE_LOOP ( 'NONE', ( #14179, #2785, #6791, #2629 ) ) ;
#14236=PLANE ( 'NONE',  #11508 ) ;
#14238=CARTESIAN_POINT ( 'NONE',  ( -31.66708739526795924, 120.0000000000000284, 5.500000000000000000 ) ) ;
#14337=ORIENTED_EDGE ( 'NONE', *, *, #15468, .T. ) ;
#14367=( GEOMETRIC_REPRESENTATION_CONTEXT ( 3 ) GLOBAL_UNCERTAINTY_ASSIGNED_CONTEXT ( ( #3789 ) ) GLOBAL_UNIT_ASSIGNED_CONTEXT ( ( #696, #13980, #2099 ) ) REPRESENTATION_CONTEXT ( 'NONE', 'WORKASPACE' ) );
#14393=CARTESIAN_POINT ( 'NONE',  ( -31.66708739526795924, 101.0000000000000142, -5.500000000000000000 ) ) ;
#14410=EDGE_CURVE ( 'NONE', #3475, #10732, #16135, .T. ) ;
#14588=ORIENTED_EDGE ( 'NONE', *, *, #6752, .T. ) ;
#14648=AXIS2_PLACEMENT_3D ( 'NONE', #1501, #4332, #16552 ) ;
#14672=CARTESIAN_POINT ( 'NONE',  ( -32.65377812985506978, 100.8098204658883361, -4.906772862994290385 ) ) ;
#14682=AXIS2_PLACEMENT_3D ( 'NONE', #8120, #13532, #16110 ) ;
#14684=VECTOR ( 'NONE', #11872, 1000.000000000000000 ) ;
#14879=CIRCLE ( 'NONE', #7245, 1.000000000000000888 ) ;
#14921=DIRECTION ( 'NONE',  ( -0.000000000000000000, 0.000000000000000000, -1.000000000000000000 ) ) ;
#14962=EDGE_LOOP ( 'NONE', ( #14337, #17167, #10940, #13213 ) ) ;
#14975=ORIENTED_EDGE ( 'NONE', *, *, #155, .F. ) ;
#15016=FACE_OUTER_BOUND ( 'NONE', #1792, .T. ) ;
#15090=VERTEX_POINT ( 'NONE', #12775 ) ;
#15121=CARTESIAN_POINT ( 'NONE',  ( -32.64269715136552463, 118.7804878048780779, 5.500000000000000000 ) ) ;
#15168=AXIS2_PLACEMENT_3D ( 'NONE', #11368, #2958, #14033 ) ;
#15170=CARTESIAN_POINT ( 'NONE',  ( -31.66708739526795924, 100.0000000000000142, 5.500000000000000000 ) ) ;
#15186=COLOUR_RGB ( '', 0.40784314, 0.44705882, 0.49803922) ;
#15187=DIRECTION ( 'NONE',  ( -0.000000000000000000, -0.000000000000000000, -1.000000000000000000 ) ) ;
#15206=CARTESIAN_POINT ( 'NONE',  ( -31.66708739526795924, 119.0000000000000284, 5.500000000000000000 ) ) ;
#15244=CARTESIAN_POINT ( 'NONE',  ( -32.59761674097720174, 119.3792650757569191, 5.080178642862611227 ) ) ;
#15266=DIRECTION ( 'NONE',  ( -0.000000000000000000, -0.000000000000000000, -1.000000000000000000 ) ) ;
#15299=AXIS2_PLACEMENT_3D ( 'NONE', #4475, #15266, #5713 ) ;
#15302=DIRECTION ( 'NONE',  ( -0.000000000000000000, 0.000000000000000000, -1.000000000000000000 ) ) ;
#15316=ORIENTED_EDGE ( 'NONE', *, *, #3285, .F. ) ;
#15324=CYLINDRICAL_SURFACE ( 'NONE', #8500, 1.000000000000000888 ) ;
#15326=EDGE_CURVE ( 'NONE', #3275, #6638, #13203, .T. ) ;
#15331=CARTESIAN_POINT ( 'NONE',  ( -32.55406425504675383, 119.4745293701281526, 5.163900856522909422 ) ) ;
#15381=SURFACE_STYLE_FILL_AREA ( #11575 ) ;
#15468=EDGE_CURVE ( 'NONE', #11430, #4227, #7054, .T. ) ;
#15564=DIRECTION ( 'NONE',  ( -1.000000000000000000, 0.000000000000000000, 0.000000000000000000 ) ) ;
#15644=SURFACE_STYLE_USAGE ( .BOTH. , #3441 ) ;
#15700=VERTEX_POINT ( 'NONE', #331 ) ;
#15717=DIRECTION ( 'NONE',  ( 1.000000000000000000, -0.000000000000000000, -0.000000000000000000 ) ) ;
#15763=B_SPLINE_CURVE_WITH_KNOTS ( 'NONE', 3,
 ( #733, #7540, #3473, #907 ),
 .UNSPECIFIED., .F., .F.,
 ( 4, 4 ),
 ( -6.324563032112924020E-06, 0.0003067249959486639528 ),
 .UNSPECIFIED. ) ;
#15886=B_SPLINE_CURVE_WITH_KNOTS ( 'NONE', 3,
 ( #5018, #7671, #6531, #17236, #3973, #9085, #11918, #14672, #11733, #10410 ),
 .UNSPECIFIED., .F., .F.,
 ( 4, 2, 2, 2, 4 ),
 ( 0.000000000000000000, 0.0003951437508621859934, 0.0007902875017243719867, 0.001185431252586558034, 0.001580575003448743973 ),
 .UNSPECIFIED. ) ;
#15955=CARTESIAN_POINT ( 'NONE',  ( -32.64269715136552463, 101.2195121951219647, 4.500000000000000000 ) ) ;
#15963=ORIENTED_EDGE ( 'NONE', *, *, #2784, .T. ) ;
#16009=UNCERTAINTY_MEASURE_WITH_UNIT (LENGTH_MEASURE( 1.000000000000000082E-05 ), #6009, 'distance_accuracy_value', 'NONE');
#16050=ORIENTED_EDGE ( 'NONE', *, *, #623, .F. ) ;
#16079=VECTOR ( 'NONE', #7977, 1000.000000000000000 ) ;
#16110=DIRECTION ( 'NONE',  ( 0.000000000000000000, 0.000000000000000000, 1.000000000000000000 ) ) ;
#16113=VECTOR ( 'NONE', #2186, 1000.000000000000000 ) ;
#16135=LINE ( 'NONE', #8149, #16079 ) ;
#16154=EDGE_LOOP ( 'NONE', ( #6111, #528, #13088, #9645 ) ) ;
#16191=B_SPLINE_CURVE_WITH_KNOTS ( 'NONE', 3,
 ( #12033, #13367, #6640, #2744, #12386, #4249, #1500, #10964, #8223, #2828 ),
 .UNSPECIFIED., .F., .F.,
 ( 4, 2, 2, 2, 4 ),
 ( 6.992893892674702526E-18, 0.0003951437508572265816, 0.0007902875017144461159, 0.001185431252571665650, 0.001580575003428885293 ),
 .UNSPECIFIED. ) ;
#16193=ORIENTED_EDGE ( 'NONE', *, *, #13896, .T. ) ;
#16308=ORIENTED_EDGE ( 'NONE', *, *, #6752, .F. ) ;
#16378=EDGE_CURVE ( 'NONE', #3275, #15090, #11147, .T. ) ;
#16552=DIRECTION ( 'NONE',  ( -1.000000000000000000, 2.707861035671114735E-15, 0.000000000000000000 ) ) ;
#16566=CARTESIAN_POINT ( 'NONE',  ( -24.93725393319379435, 120.0000000000000284, 5.500000000000000000 ) ) ;
#16574=CARTESIAN_POINT ( 'NONE',  ( -31.66708739526795924, 119.0000000000000284, 5.500000000000000000 ) ) ;
#16587=CARTESIAN_POINT ( 'NONE',  ( -32.64269715136552463, 118.7804878048780779, -4.499999999999999112 ) ) ;
#16620=ORIENTED_EDGE ( 'NONE', *, *, #9112, .F. ) ;
#16631=ORIENTED_EDGE ( 'NONE', *, *, #15468, .F. ) ;
#16707=CIRCLE ( 'NONE', #4833, 1.000000000000000888 ) ;
#16773=DIRECTION ( 'NONE',  ( -1.000000000000000000, -3.469446951953614189E-16, 0.000000000000000000 ) ) ;
#16838=ORIENTED_EDGE ( 'NONE', *, *, #3285, .T. ) ;
#16849=ADVANCED_FACE ( 'NONE', ( #11221 ), #14236, .T. ) ;
#16854=PLANE ( 'NONE',  #13031 ) ;
#16864=CARTESIAN_POINT ( 'NONE',  ( -32.66708739526796990, 100.9060348297503538, 4.814896201975309431 ) ) ;
#16890=EDGE_CURVE ( 'NONE', #17452, #10732, #15886, .T. ) ;
#16900=MANIFOLD_SOLID_BREP ( 'Fillet1', #9783 ) ;
#16949=AXIS2_PLACEMENT_3D ( 'NONE', #2668, #2759, #1168 ) ;
#17019=ADVANCED_FACE ( 'NONE', ( #15016 ), #11115, .F. ) ;
#17050=CARTESIAN_POINT ( 'NONE',  ( -24.93725393319379435, 120.0000000000000284, -5.500000000000000000 ) ) ;
#17058=EDGE_LOOP ( 'NONE', ( #9448, #16620, #13318, #9343 ) ) ;
#17123=DIRECTION ( 'NONE',  ( -0.000000000000000000, -0.000000000000000000, -1.000000000000000000 ) ) ;
#17132=CARTESIAN_POINT ( 'NONE',  ( -32.93725393319379435, 120.0000000000000284, -5.500000000000000000 ) ) ;
#17167=ORIENTED_EDGE ( 'NONE', *, *, #12849, .T. ) ;
#17183=ORIENTED_EDGE ( 'NONE', *, *, #1979, .F. ) ;
#17236=CARTESIAN_POINT ( 'NONE',  ( -32.34996859905194810, 100.2591029109095189, -5.378151393592372820 ) ) ;
#17295=EDGE_LOOP ( 'NONE', ( #7402, #764, #7169, #2404, #178, #5741 ) ) ;
#17305=UNCERTAINTY_MEASURE_WITH_UNIT (LENGTH_MEASURE( 1.000000000000000082E-05 ), #11826, 'distance_accuracy_value', 'NONE');
#17341=VERTEX_POINT ( 'NONE', #5782 ) ;
#17423=FACE_OUTER_BOUND ( 'NONE', #16154, .T. ) ;
#17452=VERTEX_POINT ( 'NONE', #2381 ) ;
ENDSEC;
END-ISO-10303-21;
